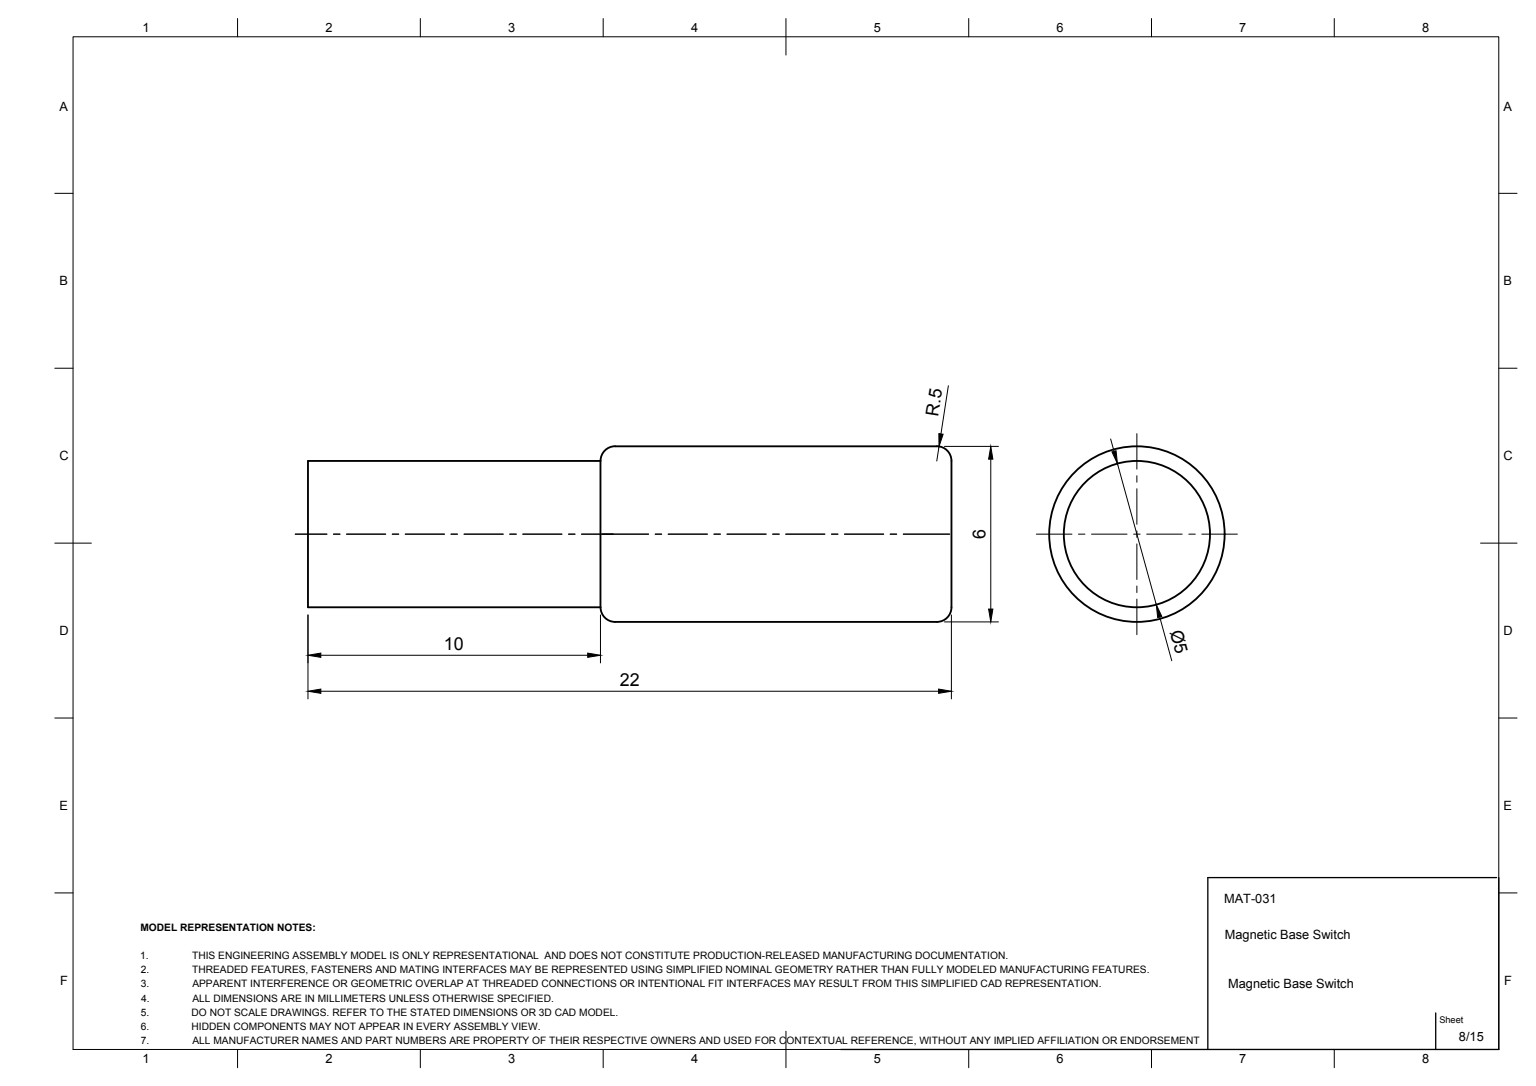
ISO-10303-21;
HEADER;
/* Generated by software containing ST-Developer
 * from STEP Tools, Inc. (www.steptools.com) 
 */

FILE_DESCRIPTION(
/* description */ ('STEP AP214'),
/* implementation_level */ '2;1');

FILE_NAME(
/* name */ 'Magnetic Base Switch.step',
/* time_stamp */ '2026-11-14T06:58:01-08:00',
/* author */ (''),
/* organization */ (''),
/* preprocessor_version */ 'ST-DEVELOPER v20.2',
/* originating_system */ 'Autodesk Translation Framework v15.17.0.0',
/* authorisation */ '');

FILE_SCHEMA (('AUTOMOTIVE_DESIGN { 1 0 10303 214 3 1 1 }'));
ENDSEC;

DATA;
#10=MECHANICAL_DESIGN_GEOMETRIC_PRESENTATION_REPRESENTATION('',(#1151),#38635);
#142=TOROIDAL_SURFACE('',#18022,2.5,0.5);
#143=TOROIDAL_SURFACE('',#18027,2.5,0.5);
#1117=SHAPE_REPRESENTATION_RELATIONSHIP('SRR','None',#38690,#1131);
#1131=ADVANCED_BREP_SHAPE_REPRESENTATION('',(#1177),#38626);
#1151=STYLED_ITEM('',(#38767),#1177);
#1177=MANIFOLD_SOLID_BREP('Body1',#17617);
#1250=PLANE('',#18034);
#1251=PLANE('',#18035);
#1792=FACE_OUTER_BOUND('',#2808,.T.);
#1793=FACE_OUTER_BOUND('',#2809,.T.);
#1794=FACE_OUTER_BOUND('',#2810,.T.);
#1795=FACE_OUTER_BOUND('',#2811,.T.);
#1796=FACE_OUTER_BOUND('',#2812,.T.);
#1797=FACE_OUTER_BOUND('',#2813,.T.);
#2808=EDGE_LOOP('',(#11649,#11650,#11651,#11652,#11653));
#2809=EDGE_LOOP('',(#11654,#11655,#11656,#11657));
#2810=EDGE_LOOP('',(#11658,#11659,#11660,#11661));
#2811=EDGE_LOOP('',(#11662,#11663,#11664,#11665,#11666));
#2812=EDGE_LOOP('',(#11667));
#2813=EDGE_LOOP('',(#11668));
#3877=LINE('',#29934,#4821);
#3878=LINE('',#29937,#4822);
#4821=VECTOR('',#20412,2.5);
#4822=VECTOR('',#20417,3.);
#5667=CIRCLE('',#18023,3.);
#5668=CIRCLE('',#18024,3.);
#5669=CIRCLE('',#18025,0.5);
#5670=CIRCLE('',#18026,2.5);
#5671=CIRCLE('',#18028,3.);
#5672=CIRCLE('',#18029,0.5);
#5673=CIRCLE('',#18030,2.5);
#5674=CIRCLE('',#18032,2.5);
#6757=VERTEX_POINT('',#29919);
#6758=VERTEX_POINT('',#29920);
#6759=VERTEX_POINT('',#29923);
#6760=VERTEX_POINT('',#29927);
#6761=VERTEX_POINT('',#29929);
#6762=VERTEX_POINT('',#29933);
#8611=EDGE_CURVE('',#6757,#6758,#5667,.T.);
#8612=EDGE_CURVE('',#6758,#6757,#5668,.T.);
#8613=EDGE_CURVE('',#6758,#6759,#5669,.T.);
#8614=EDGE_CURVE('',#6759,#6759,#5670,.T.);
#8615=EDGE_CURVE('',#6760,#6760,#5671,.T.);
#8616=EDGE_CURVE('',#6760,#6761,#5672,.T.);
#8617=EDGE_CURVE('',#6761,#6761,#5673,.T.);
#8618=EDGE_CURVE('',#6761,#6762,#3877,.T.);
#8619=EDGE_CURVE('',#6762,#6762,#5674,.T.);
#8620=EDGE_CURVE('',#6757,#6760,#3878,.T.);
#11649=ORIENTED_EDGE('',*,*,#8611,.F.);
#11650=ORIENTED_EDGE('',*,*,#8612,.F.);
#11651=ORIENTED_EDGE('',*,*,#8613,.T.);
#11652=ORIENTED_EDGE('',*,*,#8614,.F.);
#11653=ORIENTED_EDGE('',*,*,#8613,.F.);
#11654=ORIENTED_EDGE('',*,*,#8615,.F.);
#11655=ORIENTED_EDGE('',*,*,#8616,.T.);
#11656=ORIENTED_EDGE('',*,*,#8617,.T.);
#11657=ORIENTED_EDGE('',*,*,#8616,.F.);
#11658=ORIENTED_EDGE('',*,*,#8617,.F.);
#11659=ORIENTED_EDGE('',*,*,#8618,.T.);
#11660=ORIENTED_EDGE('',*,*,#8619,.T.);
#11661=ORIENTED_EDGE('',*,*,#8618,.F.);
#11662=ORIENTED_EDGE('',*,*,#8611,.T.);
#11663=ORIENTED_EDGE('',*,*,#8612,.T.);
#11664=ORIENTED_EDGE('',*,*,#8620,.T.);
#11665=ORIENTED_EDGE('',*,*,#8615,.T.);
#11666=ORIENTED_EDGE('',*,*,#8620,.F.);
#11667=ORIENTED_EDGE('',*,*,#8614,.T.);
#11668=ORIENTED_EDGE('',*,*,#8619,.F.);
#16327=CYLINDRICAL_SURFACE('',#18031,2.5);
#16328=CYLINDRICAL_SURFACE('',#18033,3.);
#16751=ADVANCED_FACE('',(#1792),#142,.T.);
#16752=ADVANCED_FACE('',(#1793),#143,.T.);
#16753=ADVANCED_FACE('',(#1794),#16327,.T.);
#16754=ADVANCED_FACE('',(#1795),#16328,.T.);
#16755=ADVANCED_FACE('',(#1796),#1250,.F.);
#16756=ADVANCED_FACE('',(#1797),#1251,.F.);
#17617=CLOSED_SHELL('',(#16751,#16752,#16753,#16754,#16755,#16756));
#18021=AXIS2_PLACEMENT_3D('',#29917,#20390,#20391);
#18022=AXIS2_PLACEMENT_3D('',#29918,#20392,#20393);
#18023=AXIS2_PLACEMENT_3D('',#29921,#20394,#20395);
#18024=AXIS2_PLACEMENT_3D('',#29922,#20396,#20397);
#18025=AXIS2_PLACEMENT_3D('',#29924,#20398,#20399);
#18026=AXIS2_PLACEMENT_3D('',#29925,#20400,#20401);
#18027=AXIS2_PLACEMENT_3D('',#29926,#20402,#20403);
#18028=AXIS2_PLACEMENT_3D('',#29928,#20404,#20405);
#18029=AXIS2_PLACEMENT_3D('',#29930,#20406,#20407);
#18030=AXIS2_PLACEMENT_3D('',#29931,#20408,#20409);
#18031=AXIS2_PLACEMENT_3D('',#29932,#20410,#20411);
#18032=AXIS2_PLACEMENT_3D('',#29935,#20413,#20414);
#18033=AXIS2_PLACEMENT_3D('',#29936,#20415,#20416);
#18034=AXIS2_PLACEMENT_3D('',#29938,#20418,#20419);
#18035=AXIS2_PLACEMENT_3D('',#29939,#20420,#20421);
#20390=DIRECTION('axis',(0.,0.,1.));
#20391=DIRECTION('refdir',(1.,0.,0.));
#20392=DIRECTION('center_axis',(0.,0.,-1.));
#20393=DIRECTION('ref_axis',(-1.,0.,0.));
#20394=DIRECTION('center_axis',(0.,0.,-1.));
#20395=DIRECTION('ref_axis',(-1.,0.,0.));
#20396=DIRECTION('center_axis',(0.,0.,-1.));
#20397=DIRECTION('ref_axis',(-1.,0.,0.));
#20398=DIRECTION('center_axis',(-1.22464679914735E-16,-1.,0.));
#20399=DIRECTION('ref_axis',(1.,-1.22464679914735E-16,0.));
#20400=DIRECTION('center_axis',(0.,0.,1.));
#20401=DIRECTION('ref_axis',(-1.,0.,0.));
#20402=DIRECTION('center_axis',(0.,0.,1.));
#20403=DIRECTION('ref_axis',(1.,0.,0.));
#20404=DIRECTION('center_axis',(0.,0.,1.));
#20405=DIRECTION('ref_axis',(1.,0.,0.));
#20406=DIRECTION('center_axis',(1.22464679914735E-16,-1.,0.));
#20407=DIRECTION('ref_axis',(-1.,-1.22464679914735E-16,0.));
#20408=DIRECTION('center_axis',(0.,0.,1.));
#20409=DIRECTION('ref_axis',(1.,0.,0.));
#20410=DIRECTION('center_axis',(0.,0.,1.));
#20411=DIRECTION('ref_axis',(1.,0.,0.));
#20412=DIRECTION('',(0.,0.,-1.));
#20413=DIRECTION('center_axis',(0.,0.,1.));
#20414=DIRECTION('ref_axis',(1.,0.,0.));
#20415=DIRECTION('center_axis',(0.,0.,1.));
#20416=DIRECTION('ref_axis',(1.,0.,0.));
#20417=DIRECTION('',(0.,0.,-1.));
#20418=DIRECTION('center_axis',(0.,0.,-1.));
#20419=DIRECTION('ref_axis',(-1.,0.,0.));
#20420=DIRECTION('center_axis',(0.,0.,1.));
#20421=DIRECTION('ref_axis',(1.,0.,0.));
#29917=CARTESIAN_POINT('',(0.,0.,0.));
#29918=CARTESIAN_POINT('Origin',(0.,0.,-0.5));
#29919=CARTESIAN_POINT('',(-3.,3.67394039744206E-16,-0.5));
#29920=CARTESIAN_POINT('',(3.,-3.67394039744206E-16,-0.5));
#29921=CARTESIAN_POINT('Origin',(0.,0.,-0.5));
#29922=CARTESIAN_POINT('Origin',(0.,0.,-0.5));
#29923=CARTESIAN_POINT('',(2.5,-3.06161699786838E-16,0.));
#29924=CARTESIAN_POINT('Origin',(2.5,-3.06161699786838E-16,-0.5));
#29925=CARTESIAN_POINT('Origin',(0.,0.,0.));
#29926=CARTESIAN_POINT('Origin',(0.,0.,-11.5));
#29927=CARTESIAN_POINT('',(-3.,-3.67394039744206E-16,-11.5));
#29928=CARTESIAN_POINT('Origin',(0.,0.,-11.5));
#29929=CARTESIAN_POINT('',(-2.5,-3.06161699786838E-16,-12.));
#29930=CARTESIAN_POINT('Origin',(-2.5,-3.06161699786838E-16,-11.5));
#29931=CARTESIAN_POINT('Origin',(0.,0.,-12.));
#29932=CARTESIAN_POINT('Origin',(0.,0.,0.));
#29933=CARTESIAN_POINT('',(-2.5,-3.06161699786838E-16,-22.));
#29934=CARTESIAN_POINT('',(-2.5,-3.06161699786838E-16,0.));
#29935=CARTESIAN_POINT('Origin',(0.,0.,-22.));
#29936=CARTESIAN_POINT('Origin',(0.,0.,0.));
#29937=CARTESIAN_POINT('',(-3.,-3.67394039744206E-16,0.));
#29938=CARTESIAN_POINT('Origin',(0.,0.,0.));
#29939=CARTESIAN_POINT('Origin',(0.,2.5,-22.));
#38610=UNCERTAINTY_MEASURE_WITH_UNIT(LENGTH_MEASURE(0.01),#38636,
'DISTANCE_ACCURACY_VALUE',
'Maximum model space distance between geometric entities at asserted c
onnectivities');
#38619=UNCERTAINTY_MEASURE_WITH_UNIT(LENGTH_MEASURE(0.01),#38636,
'DISTANCE_ACCURACY_VALUE',
'Maximum model space distance between geometric entities at asserted c
onnectivities');
#38626=(
GEOMETRIC_REPRESENTATION_CONTEXT(3)
GLOBAL_UNCERTAINTY_ASSIGNED_CONTEXT((#38610))
GLOBAL_UNIT_ASSIGNED_CONTEXT((#38636,#38638,#38639))
REPRESENTATION_CONTEXT('','3D')
);
#38635=(
GEOMETRIC_REPRESENTATION_CONTEXT(3)
GLOBAL_UNCERTAINTY_ASSIGNED_CONTEXT((#38619))
GLOBAL_UNIT_ASSIGNED_CONTEXT((#38636,#38638,#38639))
REPRESENTATION_CONTEXT('','3D')
);
#38636=(
LENGTH_UNIT()
NAMED_UNIT(*)
SI_UNIT(.MILLI.,.METRE.)
);
#38638=(
NAMED_UNIT(*)
PLANE_ANGLE_UNIT()
SI_UNIT($,.RADIAN.)
);
#38639=(
NAMED_UNIT(*)
SI_UNIT($,.STERADIAN.)
SOLID_ANGLE_UNIT()
);
#38646=SHAPE_DEFINITION_REPRESENTATION(#38661,#38690);
#38661=PRODUCT_DEFINITION_SHAPE('',$,#38706);
#38690=SHAPE_REPRESENTATION('',(#18021),#38626);
#38699=PRODUCT_DEFINITION_CONTEXT('part definition',#38746,'design');
#38706=PRODUCT_DEFINITION('Magnetic Base Switch','Magnetic Base Switch',
#38721,#38699);
#38721=PRODUCT_DEFINITION_FORMATION('',$,#38754);
#38746=APPLICATION_CONTEXT(
'Core Data for Automotive Mechanical Design Process');
#38747=PRODUCT_CONTEXT('part definition',#38746,'mechanical');
#38754=PRODUCT('Magnetic Base Switch','Magnetic Base Switch',$,(#38747));
#38767=PRESENTATION_STYLE_ASSIGNMENT((#38774));
#38774=SURFACE_STYLE_USAGE(.BOTH.,#38781);
#38781=SURFACE_SIDE_STYLE('',(#38788));
#38788=SURFACE_STYLE_FILL_AREA(#38795);
#38795=FILL_AREA_STYLE('Opaque(97,158,199)',(#38802));
#38802=FILL_AREA_STYLE_COLOUR('Opaque(97,158,199)',#38809);
#38809=COLOUR_RGB('Opaque(97,158,199)',0.380392156862745,0.619607843137255,
0.780392156862745);
ENDSEC;
END-ISO-10303-21;
